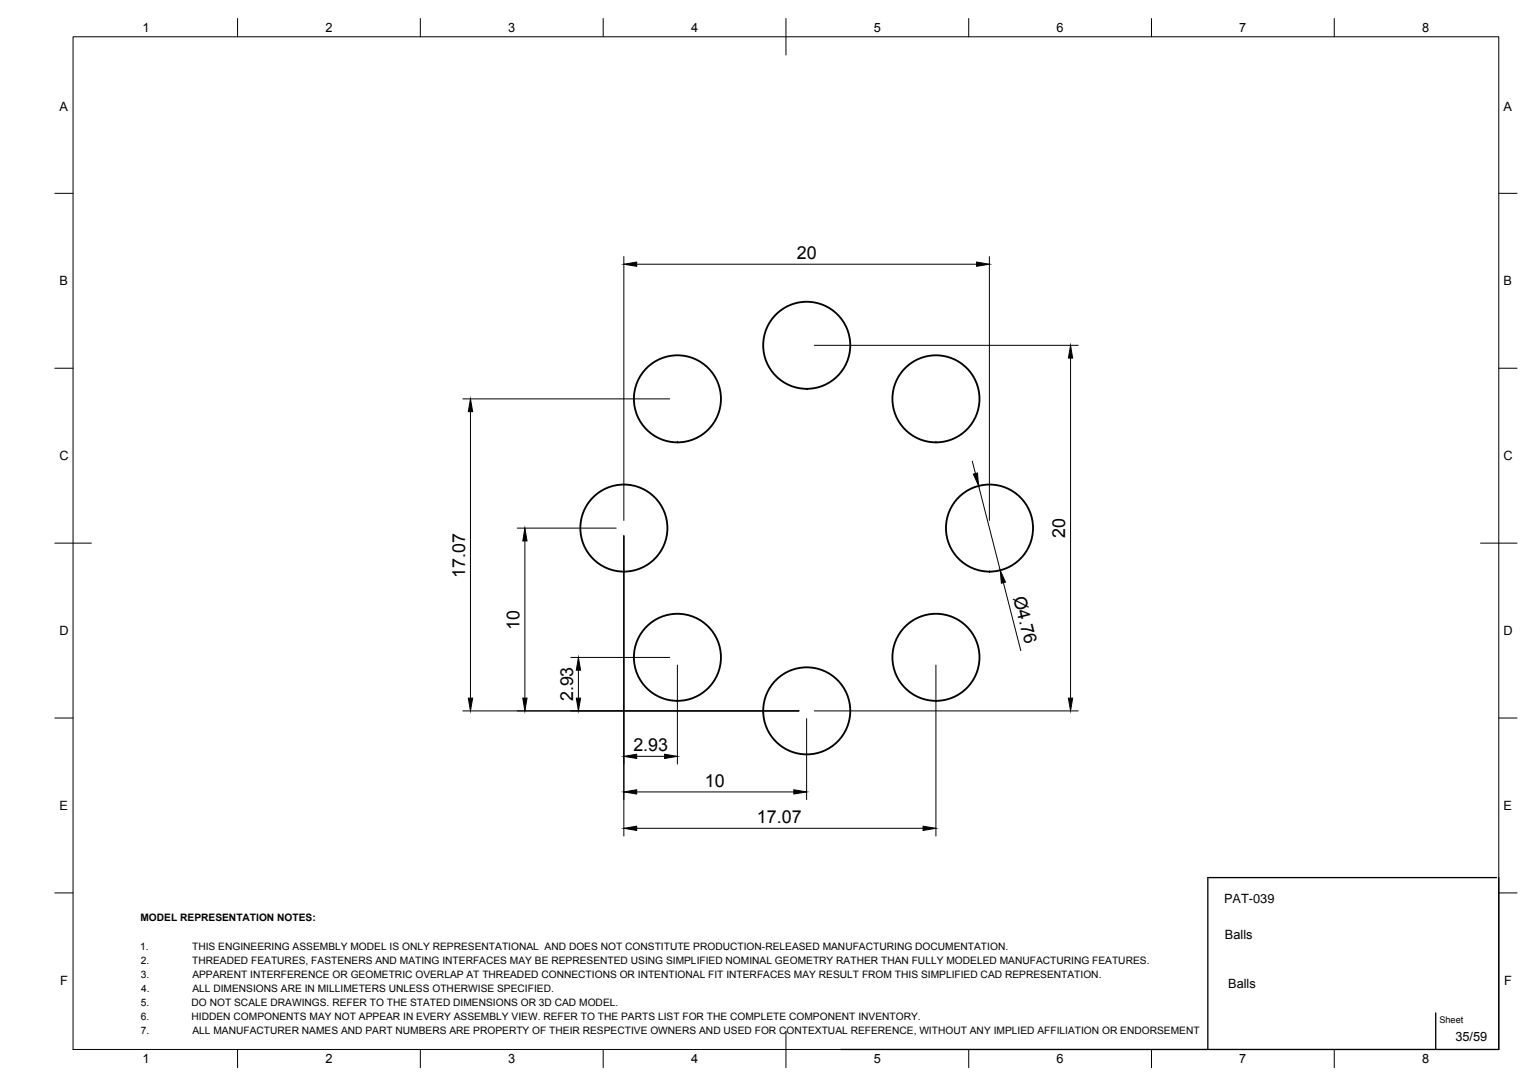
ISO-10303-21;
HEADER;
/* Generated by software containing ST-Developer
 * from STEP Tools, Inc. (www.steptools.com) 
 */

FILE_DESCRIPTION(
/* description */ ('Four-bar parallelogram arm'),
/* implementation_level */ '2;1');

FILE_NAME(
/* name */ 'Balls.step',
/* time_stamp */ '2026-10-28T03:24:55-07:00',
/* author */ (''),
/* organization */ (''),
/* preprocessor_version */ 'ST-DEVELOPER v20.2',
/* originating_system */ 'Autodesk Translation Framework v15.17.0.0',
/* authorisation */ '');

FILE_SCHEMA (('AUTOMOTIVE_DESIGN { 1 0 10303 214 3 1 1 }'));
ENDSEC;

DATA;
#10=MECHANICAL_DESIGN_GEOMETRIC_PRESENTATION_REPRESENTATION('',(#656,#657,#658,#659,#660,#661,#662,#663),#14512);
#459=SPHERICAL_SURFACE('',#8548,0.23815);
#460=SPHERICAL_SURFACE('',#8550,0.23815);
#461=SPHERICAL_SURFACE('',#8552,0.23815);
#462=SPHERICAL_SURFACE('',#8554,0.23815);
#463=SPHERICAL_SURFACE('',#8556,0.23815);
#464=SPHERICAL_SURFACE('',#8558,0.23815);
#465=SPHERICAL_SURFACE('',#8560,0.23815);
#466=SPHERICAL_SURFACE('',#8562,0.23815);
#556=SHAPE_REPRESENTATION_RELATIONSHIP('SRR','None',#14780,#606);
#606=ADVANCED_BREP_SHAPE_REPRESENTATION('',(#713,#714,#715,#716,#717,#718,
#719,#720),#14495);
#656=STYLED_ITEM('',(#15087),#713);
#657=STYLED_ITEM('',(#15087),#714);
#658=STYLED_ITEM('',(#15087),#715);
#659=STYLED_ITEM('',(#15087),#716);
#660=STYLED_ITEM('',(#15087),#717);
#661=STYLED_ITEM('',(#15087),#718);
#662=STYLED_ITEM('',(#15087),#719);
#663=STYLED_ITEM('',(#15087),#720);
#713=MANIFOLD_SOLID_BREP('Body1',#7361);
#714=MANIFOLD_SOLID_BREP('Body2',#7362);
#715=MANIFOLD_SOLID_BREP('Body3',#7363);
#716=MANIFOLD_SOLID_BREP('Body4',#7364);
#717=MANIFOLD_SOLID_BREP('Body5',#7365);
#718=MANIFOLD_SOLID_BREP('Body6',#7366);
#719=MANIFOLD_SOLID_BREP('Body7',#7367);
#720=MANIFOLD_SOLID_BREP('Body8',#7368);
#1476=FACE_OUTER_BOUND('',#2102,.T.);
#1477=FACE_OUTER_BOUND('',#2103,.T.);
#1478=FACE_OUTER_BOUND('',#2104,.T.);
#1479=FACE_OUTER_BOUND('',#2105,.T.);
#1480=FACE_OUTER_BOUND('',#2106,.T.);
#1481=FACE_OUTER_BOUND('',#2107,.T.);
#1482=FACE_OUTER_BOUND('',#2108,.T.);
#1483=FACE_OUTER_BOUND('',#2109,.T.);
#2102=EDGE_LOOP('',(#6148,#6149));
#2103=EDGE_LOOP('',(#6150,#6151));
#2104=EDGE_LOOP('',(#6152,#6153));
#2105=EDGE_LOOP('',(#6154,#6155));
#2106=EDGE_LOOP('',(#6156,#6157));
#2107=EDGE_LOOP('',(#6158,#6159));
#2108=EDGE_LOOP('',(#6160,#6161));
#2109=EDGE_LOOP('',(#6162,#6163));
#3396=CIRCLE('',#8549,0.23815);
#3397=CIRCLE('',#8551,0.23815);
#3398=CIRCLE('',#8553,0.23815);
#3399=CIRCLE('',#8555,0.23815);
#3400=CIRCLE('',#8557,0.23815);
#3401=CIRCLE('',#8559,0.23815);
#3402=CIRCLE('',#8561,0.23815);
#3403=CIRCLE('',#8563,0.23815);
#3928=VERTEX_POINT('',#13309);
#3929=VERTEX_POINT('',#13310);
#3930=VERTEX_POINT('',#13313);
#3931=VERTEX_POINT('',#13314);
#3932=VERTEX_POINT('',#13317);
#3933=VERTEX_POINT('',#13318);
#3934=VERTEX_POINT('',#13321);
#3935=VERTEX_POINT('',#13322);
#3936=VERTEX_POINT('',#13325);
#3937=VERTEX_POINT('',#13326);
#3938=VERTEX_POINT('',#13329);
#3939=VERTEX_POINT('',#13330);
#3940=VERTEX_POINT('',#13333);
#3941=VERTEX_POINT('',#13334);
#3942=VERTEX_POINT('',#13337);
#3943=VERTEX_POINT('',#13338);
#4705=EDGE_CURVE('',#3928,#3929,#3396,.T.);
#4706=EDGE_CURVE('',#3930,#3931,#3397,.T.);
#4707=EDGE_CURVE('',#3932,#3933,#3398,.T.);
#4708=EDGE_CURVE('',#3934,#3935,#3399,.T.);
#4709=EDGE_CURVE('',#3936,#3937,#3400,.T.);
#4710=EDGE_CURVE('',#3938,#3939,#3401,.T.);
#4711=EDGE_CURVE('',#3940,#3941,#3402,.T.);
#4712=EDGE_CURVE('',#3942,#3943,#3403,.T.);
#6148=ORIENTED_EDGE('',*,*,#4705,.T.);
#6149=ORIENTED_EDGE('',*,*,#4705,.F.);
#6150=ORIENTED_EDGE('',*,*,#4706,.T.);
#6151=ORIENTED_EDGE('',*,*,#4706,.F.);
#6152=ORIENTED_EDGE('',*,*,#4707,.T.);
#6153=ORIENTED_EDGE('',*,*,#4707,.F.);
#6154=ORIENTED_EDGE('',*,*,#4708,.T.);
#6155=ORIENTED_EDGE('',*,*,#4708,.F.);
#6156=ORIENTED_EDGE('',*,*,#4709,.T.);
#6157=ORIENTED_EDGE('',*,*,#4709,.F.);
#6158=ORIENTED_EDGE('',*,*,#4710,.T.);
#6159=ORIENTED_EDGE('',*,*,#4710,.F.);
#6160=ORIENTED_EDGE('',*,*,#4711,.T.);
#6161=ORIENTED_EDGE('',*,*,#4711,.F.);
#6162=ORIENTED_EDGE('',*,*,#4712,.T.);
#6163=ORIENTED_EDGE('',*,*,#4712,.F.);
#7181=ADVANCED_FACE('',(#1476),#459,.T.);
#7182=ADVANCED_FACE('',(#1477),#460,.T.);
#7183=ADVANCED_FACE('',(#1478),#461,.T.);
#7184=ADVANCED_FACE('',(#1479),#462,.T.);
#7185=ADVANCED_FACE('',(#1480),#463,.T.);
#7186=ADVANCED_FACE('',(#1481),#464,.T.);
#7187=ADVANCED_FACE('',(#1482),#465,.T.);
#7188=ADVANCED_FACE('',(#1483),#466,.T.);
#7361=CLOSED_SHELL('',(#7181));
#7362=CLOSED_SHELL('',(#7182));
#7363=CLOSED_SHELL('',(#7183));
#7364=CLOSED_SHELL('',(#7184));
#7365=CLOSED_SHELL('',(#7185));
#7366=CLOSED_SHELL('',(#7186));
#7367=CLOSED_SHELL('',(#7187));
#7368=CLOSED_SHELL('',(#7188));
#8547=AXIS2_PLACEMENT_3D('',#13307,#10466,#10467);
#8548=AXIS2_PLACEMENT_3D('',#13308,#10468,#10469);
#8549=AXIS2_PLACEMENT_3D('',#13311,#10470,#10471);
#8550=AXIS2_PLACEMENT_3D('',#13312,#10472,#10473);
#8551=AXIS2_PLACEMENT_3D('',#13315,#10474,#10475);
#8552=AXIS2_PLACEMENT_3D('',#13316,#10476,#10477);
#8553=AXIS2_PLACEMENT_3D('',#13319,#10478,#10479);
#8554=AXIS2_PLACEMENT_3D('',#13320,#10480,#10481);
#8555=AXIS2_PLACEMENT_3D('',#13323,#10482,#10483);
#8556=AXIS2_PLACEMENT_3D('',#13324,#10484,#10485);
#8557=AXIS2_PLACEMENT_3D('',#13327,#10486,#10487);
#8558=AXIS2_PLACEMENT_3D('',#13328,#10488,#10489);
#8559=AXIS2_PLACEMENT_3D('',#13331,#10490,#10491);
#8560=AXIS2_PLACEMENT_3D('',#13332,#10492,#10493);
#8561=AXIS2_PLACEMENT_3D('',#13335,#10494,#10495);
#8562=AXIS2_PLACEMENT_3D('',#13336,#10496,#10497);
#8563=AXIS2_PLACEMENT_3D('',#13339,#10498,#10499);
#10466=DIRECTION('axis',(0.,0.,1.));
#10467=DIRECTION('refdir',(1.,0.,0.));
#10468=DIRECTION('center_axis',(0.,0.,1.));
#10469=DIRECTION('ref_axis',(1.,0.,0.));
#10470=DIRECTION('center_axis',(1.22464679914735E-16,-1.,0.));
#10471=DIRECTION('ref_axis',(-1.,-1.22464679914735E-16,0.));
#10472=DIRECTION('center_axis',(0.707106781186548,0.,0.707106781186548));
#10473=DIRECTION('ref_axis',(0.707106781186548,0.,-0.707106781186548));
#10474=DIRECTION('center_axis',(8.65956056235494E-17,-1.,-8.65956056235493E-17));
#10475=DIRECTION('ref_axis',(-0.707106781186547,-1.22464679914735E-16,0.707106781186547));
#10476=DIRECTION('center_axis',(1.,0.,0.));
#10477=DIRECTION('ref_axis',(6.12323399573676E-17,0.,-1.));
#10478=DIRECTION('center_axis',(7.49879891330929E-33,-1.,-1.22464679914735E-16));
#10479=DIRECTION('ref_axis',(-6.12323399573676E-17,-1.22464679914735E-16,
1.));
#10480=DIRECTION('center_axis',(0.707106781186548,0.,-0.707106781186548));
#10481=DIRECTION('ref_axis',(-0.707106781186548,0.,-0.707106781186548));
#10482=DIRECTION('center_axis',(-8.65956056235493E-17,-1.,-8.65956056235494E-17));
#10483=DIRECTION('ref_axis',(0.707106781186547,-1.22464679914735E-16,0.707106781186547));
#10484=DIRECTION('center_axis',(0.,0.,-1.));
#10485=DIRECTION('ref_axis',(-1.,0.,-1.22464679914735E-16));
#10486=DIRECTION('center_axis',(-1.22464679914735E-16,-1.,-1.49975978266186E-32));
#10487=DIRECTION('ref_axis',(1.,-1.22464679914735E-16,1.22464679914735E-16));
#10488=DIRECTION('center_axis',(-0.707106781186547,0.,-0.707106781186548));
#10489=DIRECTION('ref_axis',(-0.707106781186548,0.,0.707106781186547));
#10490=DIRECTION('center_axis',(-8.65956056235493E-17,-1.,8.65956056235493E-17));
#10491=DIRECTION('ref_axis',(0.707106781186548,-1.22464679914735E-16,-0.707106781186547));
#10492=DIRECTION('center_axis',(-1.,0.,0.));
#10493=DIRECTION('ref_axis',(-1.83697019872103E-16,0.,1.));
#10494=DIRECTION('center_axis',(-2.24963967399279E-32,-1.,1.22464679914735E-16));
#10495=DIRECTION('ref_axis',(1.83697019872103E-16,-1.22464679914735E-16,
-1.));
#10496=DIRECTION('center_axis',(-0.707106781186548,0.,0.707106781186548));
#10497=DIRECTION('ref_axis',(0.707106781186547,0.,0.707106781186548));
#10498=DIRECTION('center_axis',(8.65956056235493E-17,-1.,8.65956056235493E-17));
#10499=DIRECTION('ref_axis',(-0.707106781186547,-1.22464679914735E-16,-0.707106781186548));
#13307=CARTESIAN_POINT('',(0.,0.,0.));
#13308=CARTESIAN_POINT('Origin',(1.,0.,0.));
#13309=CARTESIAN_POINT('',(1.,-1.78583896120461E-33,0.23815));
#13310=CARTESIAN_POINT('',(1.,-1.78583896120461E-33,-0.23815));
#13311=CARTESIAN_POINT('Origin',(1.,0.,0.));
#13312=CARTESIAN_POINT('Origin',(0.707106781186548,0.,-0.707106781186547));
#13313=CARTESIAN_POINT('',(0.875504261126124,-1.78583896120461E-33,-0.538709301246971));
#13314=CARTESIAN_POINT('',(0.538709301246971,-1.78583896120461E-33,-0.875504261126124));
#13315=CARTESIAN_POINT('Origin',(0.707106781186548,0.,-0.707106781186547));
#13316=CARTESIAN_POINT('Origin',(6.12323399573677E-17,0.,-1.));
#13317=CARTESIAN_POINT('',(0.23815,-1.78583896120461E-33,-1.));
#13318=CARTESIAN_POINT('',(-0.23815,-1.78583896120461E-33,-1.));
#13319=CARTESIAN_POINT('Origin',(6.12323399573677E-17,0.,-1.));
#13320=CARTESIAN_POINT('Origin',(-0.707106781186547,0.,-0.707106781186548));
#13321=CARTESIAN_POINT('',(-0.538709301246971,-1.78583896120461E-33,-0.875504261126124));
#13322=CARTESIAN_POINT('',(-0.875504261126124,-1.78583896120461E-33,-0.538709301246971));
#13323=CARTESIAN_POINT('Origin',(-0.707106781186547,0.,-0.707106781186548));
#13324=CARTESIAN_POINT('Origin',(-1.,0.,-1.22464679914735E-16));
#13325=CARTESIAN_POINT('',(-1.,-1.78583896120461E-33,-0.23815));
#13326=CARTESIAN_POINT('',(-1.,-1.78583896120461E-33,0.23815));
#13327=CARTESIAN_POINT('Origin',(-1.,0.,-1.22464679914735E-16));
#13328=CARTESIAN_POINT('Origin',(-0.707106781186548,0.,0.707106781186547));
#13329=CARTESIAN_POINT('',(-0.875504261126124,-7.94881478324376E-33,0.538709301246971));
#13330=CARTESIAN_POINT('',(-0.538709301246971,4.37713686083455E-33,0.875504261126124));
#13331=CARTESIAN_POINT('Origin',(-0.707106781186548,0.,0.707106781186547));
#13332=CARTESIAN_POINT('Origin',(-1.83697019872103E-16,0.,1.));
#13333=CARTESIAN_POINT('',(-0.23815,-1.78583896120461E-33,1.));
#13334=CARTESIAN_POINT('',(0.23815,-1.78583896120461E-33,1.));
#13335=CARTESIAN_POINT('Origin',(-1.83697019872103E-16,0.,1.));
#13336=CARTESIAN_POINT('Origin',(0.707106781186547,0.,0.707106781186548));
#13337=CARTESIAN_POINT('',(0.538709301246971,-4.86732687222419E-33,0.875504261126124));
#13338=CARTESIAN_POINT('',(0.875504261126124,1.29564894981497E-33,0.538709301246971));
#13339=CARTESIAN_POINT('Origin',(0.707106781186547,0.,0.707106781186548));
#14438=UNCERTAINTY_MEASURE_WITH_UNIT(LENGTH_MEASURE(0.001),#14513,
'DISTANCE_ACCURACY_VALUE',
'Maximum model space distance between geometric entities at asserted c
onnectivities');
#14455=UNCERTAINTY_MEASURE_WITH_UNIT(LENGTH_MEASURE(0.001),#14513,
'DISTANCE_ACCURACY_VALUE',
'Maximum model space distance between geometric entities at asserted c
onnectivities');
#14495=(
GEOMETRIC_REPRESENTATION_CONTEXT(3)
GLOBAL_UNCERTAINTY_ASSIGNED_CONTEXT((#14438))
GLOBAL_UNIT_ASSIGNED_CONTEXT((#14513,#14515,#14516))
REPRESENTATION_CONTEXT('','3D')
);
#14512=(
GEOMETRIC_REPRESENTATION_CONTEXT(3)
GLOBAL_UNCERTAINTY_ASSIGNED_CONTEXT((#14455))
GLOBAL_UNIT_ASSIGNED_CONTEXT((#14513,#14515,#14516))
REPRESENTATION_CONTEXT('','3D')
);
#14513=(
LENGTH_UNIT()
NAMED_UNIT(*)
SI_UNIT(.CENTI.,.METRE.)
);
#14515=(
NAMED_UNIT(*)
PLANE_ANGLE_UNIT()
SI_UNIT($,.RADIAN.)
);
#14516=(
NAMED_UNIT(*)
SI_UNIT($,.STERADIAN.)
SOLID_ANGLE_UNIT()
);
#14556=SHAPE_DEFINITION_REPRESENTATION(#14612,#14780);
#14612=PRODUCT_DEFINITION_SHAPE('',$,#14837);
#14780=SHAPE_REPRESENTATION('',(#8547),#14495);
#14797=PRODUCT_DEFINITION_CONTEXT('part definition',#14967,'design');
#14837=PRODUCT_DEFINITION('Balls','Balls',#14893,#14797);
#14893=PRODUCT_DEFINITION_FORMATION('',$,#15008);
#14967=APPLICATION_CONTEXT(
'Core Data for Automotive Mechanical Design Process');
#14968=PRODUCT_CONTEXT('part definition',#14967,'mechanical');
#15008=PRODUCT('Balls','Balls','Balls',(#14968));
#15081=COLOUR_RGB('Grey',0.48,0.52,0.57);
#15082=FILL_AREA_STYLE_COLOUR('',#15081);
#15083=FILL_AREA_STYLE('',(#15082));
#15084=SURFACE_STYLE_FILL_AREA(#15083);
#15085=SURFACE_SIDE_STYLE('',(#15084));
#15086=SURFACE_STYLE_USAGE(.BOTH.,#15085);
#15087=PRESENTATION_STYLE_ASSIGNMENT((#15086));
ENDSEC;
END-ISO-10303-21;
